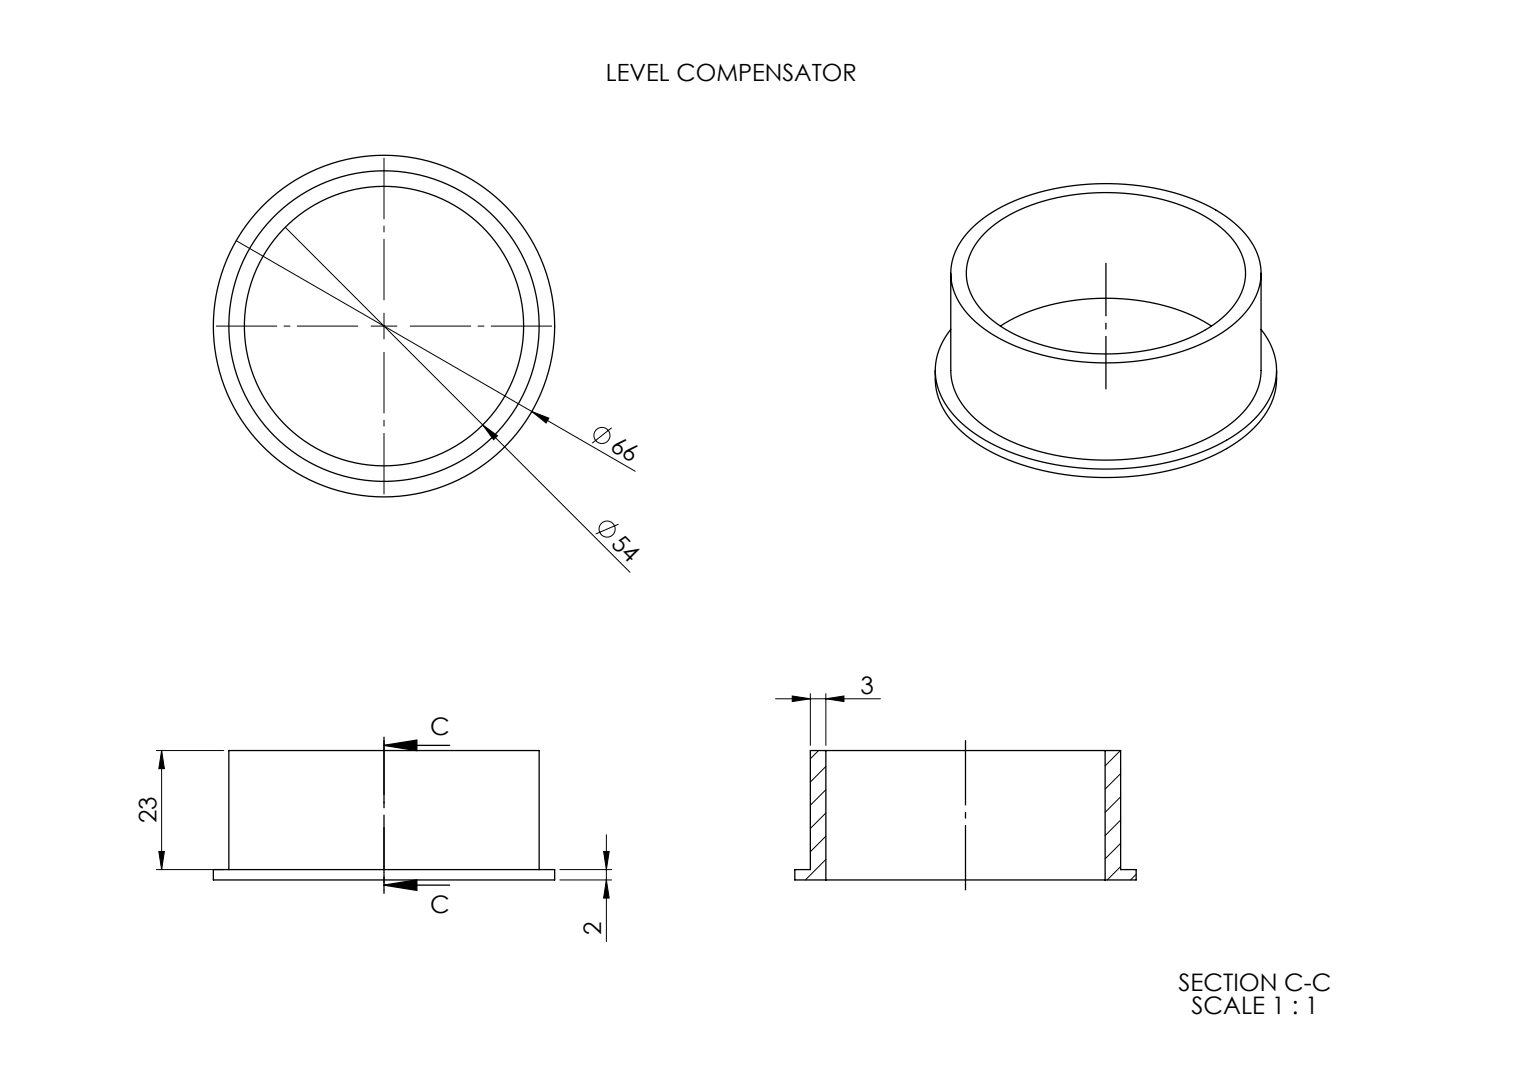
ISO-10303-21;
HEADER;
FILE_DESCRIPTION (('STEP AP214'),
    '1' );
FILE_NAME ('level compensator.step',
    '2026-10-02T18:08:48',
    ( '' ),
    ( '' ),
    'SwSTEP 2.0',
    'SolidWorks 2026',
    '' );
FILE_SCHEMA (( 'AUTOMOTIVE_DESIGN' ));
ENDSEC;

DATA;
#56=LINE ( 'NONE', #23253, #28638 ) ;
#123=ADVANCED_FACE ( 'NONE', ( #17350, #12018 ), #22832, .T. ) ;
#373=ORIENTED_EDGE ( 'NONE', *, *, #30700, .F. ) ;
#395=ORIENTED_EDGE ( 'NONE', *, *, #27322, .F. ) ;
#589=VECTOR ( 'NONE', #16460, 1000.000000000000000 ) ;
#693=CARTESIAN_POINT ( 'NONE',  ( 0.000000000000000000, -10.99999999999999645, 30.00000000000000000 ) ) ;
#907=CARTESIAN_POINT ( 'NONE',  ( 0.000000000000000000, -12.99999999999999822, 0.000000000000000000 ) ) ;
#1030=EDGE_CURVE ( 'NONE', #9545, #23066, #12266, .T. ) ;
#1166=AXIS2_PLACEMENT_3D ( 'NONE', #29236, #16220, #24104 ) ;
#1349=CARTESIAN_POINT ( 'NONE',  ( 4.041334437186266200E-15, -10.99999999999999645, 33.00000000000000000 ) ) ;
#1374=DIRECTION ( 'NONE',  ( 0.000000000000000000, -1.000000000000000000, 0.000000000000000000 ) ) ;
#1376=AXIS2_PLACEMENT_3D ( 'NONE', #6186, #27460, #21818 ) ;
#1489=CARTESIAN_POINT ( 'NONE',  ( 0.000000000000000000, 11.99999999999999645, 30.00000000000000000 ) ) ;
#1689=EDGE_CURVE ( 'NONE', #7405, #23066, #10874, .T. ) ;
#1782=EDGE_CURVE ( 'NONE', #20971, #6049, #18351, .T. ) ;
#1786=CARTESIAN_POINT ( 'NONE',  ( 4.041334437186266200E-15, -12.99999999999999822, 33.00000000000000000 ) ) ;
#1877=( LENGTH_UNIT ( ) NAMED_UNIT ( * ) SI_UNIT ( .MILLI., .METRE. ) );
#1908=ORIENTED_EDGE ( 'NONE', *, *, #1030, .T. ) ;
#1920=COLOUR_RGB ( '', 0.66274510, 0.83137255, 0.94901961) ;
#2047=FACE_BOUND ( 'NONE', #31107, .T. ) ;
#2135=DIRECTION ( 'NONE',  ( 0.000000000000000000, -1.000000000000000000, 0.000000000000000000 ) ) ;
#2140=DIRECTION ( 'NONE',  ( 0.000000000000000000, -1.000000000000000000, 0.000000000000000000 ) ) ;
#2313=DIRECTION ( 'NONE',  ( 0.000000000000000000, 0.000000000000000000, 1.000000000000000000 ) ) ;
#2455=ORIENTED_EDGE ( 'NONE', *, *, #27322, .T. ) ;
#2485=CYLINDRICAL_SURFACE ( 'NONE', #26189, 30.00000000000000000 ) ;
#2562=EDGE_LOOP ( 'NONE', ( #9167, #24597 ) ) ;
#2645=EDGE_LOOP ( 'NONE', ( #22385, #6844, #9366, #19276 ) ) ;
#2667=ADVANCED_FACE ( 'NONE', ( #20423, #2047 ), #4449, .F. ) ;
#2692=VERTEX_POINT ( 'NONE', #30872 ) ;
#2999=FACE_OUTER_BOUND ( 'NONE', #2645, .T. ) ;
#3170=CYLINDRICAL_SURFACE ( 'NONE', #1166, 27.00000000000000000 ) ;
#3270=ORIENTED_EDGE ( 'NONE', *, *, #13968, .F. ) ;
#3340=ADVANCED_FACE ( 'NONE', ( #23256 ), #2485, .T. ) ;
#3476=CARTESIAN_POINT ( 'NONE',  ( 0.000000000000000000, -10.99999999999999645, 0.000000000000000000 ) ) ;
#3549=DIRECTION ( 'NONE',  ( 0.000000000000000000, 0.000000000000000000, -1.000000000000000000 ) ) ;
#3597=MECHANICAL_DESIGN_GEOMETRIC_PRESENTATION_REPRESENTATION('',(#10711),#7987);
#3804=EDGE_CURVE ( 'NONE', #2692, #30646, #17443, .T. ) ;
#3810=DIRECTION ( 'NONE',  ( 0.000000000000000000, -1.000000000000000000, 0.000000000000000000 ) ) ;
#3928=AXIS2_PLACEMENT_3D ( 'NONE', #4887, #4714, #2313 ) ;
#4023=CARTESIAN_POINT ( 'NONE',  ( 0.000000000000000000, 11.99999999999999645, 0.000000000000000000 ) ) ;
#4037=CIRCLE ( 'NONE', #16120, 33.00000000000000000 ) ;
#4449=PLANE ( 'NONE',  #17391 ) ;
#4469=EDGE_LOOP ( 'NONE', ( #23792, #1908 ) ) ;
#4548=DIRECTION ( 'NONE',  ( 0.000000000000000000, 0.000000000000000000, -1.000000000000000000 ) ) ;
#4605=FACE_BOUND ( 'NONE', #20807, .T. ) ;
#4714=DIRECTION ( 'NONE',  ( -0.000000000000000000, 1.000000000000000000, -0.000000000000000000 ) ) ;
#4884=CARTESIAN_POINT ( 'NONE',  ( 0.000000000000000000, -12.99999999999999822, 0.000000000000000000 ) ) ;
#4887=CARTESIAN_POINT ( 'NONE',  ( 0.000000000000000000, -12.99999999999999822, 0.000000000000000000 ) ) ;
#4955=EDGE_CURVE ( 'NONE', #6049, #20971, #26216, .T. ) ;
#5149=CLOSED_SHELL ( 'NONE', ( #16079, #9447, #29369, #3340, #123, #2667, #9646, #28558, #31037 ) ) ;
#5223=ORIENTED_EDGE ( 'NONE', *, *, #1782, .F. ) ;
#5228=FACE_OUTER_BOUND ( 'NONE', #11535, .T. ) ;
#5566=DIRECTION ( 'NONE',  ( -0.000000000000000000, 1.000000000000000000, -0.000000000000000000 ) ) ;
#5696=AXIS2_PLACEMENT_3D ( 'NONE', #28118, #27437, #33431 ) ;
#6011=ORIENTED_EDGE ( 'NONE', *, *, #25422, .F. ) ;
#6033=DIRECTION ( 'NONE',  ( 0.000000000000000000, -1.000000000000000000, 0.000000000000000000 ) ) ;
#6049=VERTEX_POINT ( 'NONE', #17755 ) ;
#6163=PRODUCT_DEFINITION ( 'UNKNOWN', '', #13174, #6504 ) ;
#6186=CARTESIAN_POINT ( 'NONE',  ( 0.000000000000000000, 0.000000000000000000, 0.000000000000000000 ) ) ;
#6249=CIRCLE ( 'NONE', #27606, 30.00000000000000000 ) ;
#6504=PRODUCT_DEFINITION_CONTEXT ( 'detailed design', #21934, 'design' ) ;
#6669=DIRECTION ( 'NONE',  ( 1.000000000000000000, 0.000000000000000000, 0.000000000000000000 ) ) ;
#6844=ORIENTED_EDGE ( 'NONE', *, *, #28947, .T. ) ;
#6912=ORIENTED_EDGE ( 'NONE', *, *, #14411, .T. ) ;
#7039=VERTEX_POINT ( 'NONE', #1349 ) ;
#7285=FACE_OUTER_BOUND ( 'NONE', #32956, .T. ) ;
#7321=CIRCLE ( 'NONE', #29774, 27.00000000000000000 ) ;
#7376=SURFACE_SIDE_STYLE ('',( #10130 ) ) ;
#7405=VERTEX_POINT ( 'NONE', #23151 ) ;
#7541=DIRECTION ( 'NONE',  ( 0.000000000000000000, -0.000000000000000000, -1.000000000000000000 ) ) ;
#7828=EDGE_LOOP ( 'NONE', ( #373, #24739 ) ) ;
#7973=CARTESIAN_POINT ( 'NONE',  ( 0.000000000000000000, -12.99999999999999822, 0.000000000000000000 ) ) ;
#7987=( GEOMETRIC_REPRESENTATION_CONTEXT ( 3 ) GLOBAL_UNCERTAINTY_ASSIGNED_CONTEXT ( ( #18089 ) ) GLOBAL_UNIT_ASSIGNED_CONTEXT ( ( #1877, #9779, #20430 ) ) REPRESENTATION_CONTEXT ( 'NONE', 'WORKASPACE' ) );
#8140=( NAMED_UNIT ( * ) SI_UNIT ( $, .STERADIAN. ) SOLID_ANGLE_UNIT ( ) );
#8214=EDGE_CURVE ( 'NONE', #30646, #2692, #32934, .T. ) ;
#8281=DIRECTION ( 'NONE',  ( 0.000000000000000000, -1.000000000000000000, 0.000000000000000000 ) ) ;
#8289=ORIENTED_EDGE ( 'NONE', *, *, #30841, .T. ) ;
#8312=COLOUR_RGB ( '', 0.66274510, 0.83137255, 0.94901961) ;
#8662=ORIENTED_EDGE ( 'NONE', *, *, #1689, .F. ) ;
#8792=VERTEX_POINT ( 'NONE', #1489 ) ;
#8835=ORIENTED_EDGE ( 'NONE', *, *, #16099, .F. ) ;
#9133=AXIS2_PLACEMENT_3D ( 'NONE', #22331, #18929, #16352 ) ;
#9167=ORIENTED_EDGE ( 'NONE', *, *, #30966, .F. ) ;
#9234=CARTESIAN_POINT ( 'NONE',  ( 0.000000000000000000, -10.99999999999999645, 0.000000000000000000 ) ) ;
#9366=ORIENTED_EDGE ( 'NONE', *, *, #21542, .T. ) ;
#9369=ORIENTED_EDGE ( 'NONE', *, *, #1782, .T. ) ;
#9447=ADVANCED_FACE ( 'NONE', ( #7285 ), #17769, .F. ) ;
#9471=VECTOR ( 'NONE', #33843, 1000.000000000000000 ) ;
#9545=VERTEX_POINT ( 'NONE', #1786 ) ;
#9552=MANIFOLD_SOLID_BREP ( 'Extrude-Thin2', #5149 ) ;
#9646=ADVANCED_FACE ( 'NONE', ( #2999 ), #3170, .F. ) ;
#9683=CIRCLE ( 'NONE', #9133, 30.00000000000000000 ) ;
#9779=( NAMED_UNIT ( * ) PLANE_ANGLE_UNIT ( ) SI_UNIT ( $, .RADIAN. ) );
#9792=CARTESIAN_POINT ( 'NONE',  ( 0.000000000000000000, -12.99999999999999822, 0.000000000000000000 ) ) ;
#9928=DIRECTION ( 'NONE',  ( 0.000000000000000000, -1.000000000000000000, 0.000000000000000000 ) ) ;
#10130=SURFACE_STYLE_FILL_AREA ( #20612 ) ;
#10193=UNCERTAINTY_MEASURE_WITH_UNIT (LENGTH_MEASURE( 1.000000000000000082E-05 ), #10720, 'distance_accuracy_value', 'NONE');
#10380=CYLINDRICAL_SURFACE ( 'NONE', #33589, 33.00000000000000000 ) ;
#10448=PRODUCT_DEFINITION_SHAPE ( 'NONE', 'NONE',  #6163 ) ;
#10711=STYLED_ITEM ( 'NONE', ( #17860 ), #22997 ) ;
#10720=( LENGTH_UNIT ( ) NAMED_UNIT ( * ) SI_UNIT ( .MILLI., .METRE. ) );
#10750=ORIENTED_EDGE ( 'NONE', *, *, #8214, .T. ) ;
#10874=LINE ( 'NONE', #33873, #22682 ) ;
#11303=CARTESIAN_POINT ( 'NONE',  ( 0.000000000000000000, -12.99999999999999822, 27.00000000000000000 ) ) ;
#11535=EDGE_LOOP ( 'NONE', ( #395, #8289, #29593, #27174 ) ) ;
#11648=CARTESIAN_POINT ( 'NONE',  ( 0.000000000000000000, -12.99999999999999822, 0.000000000000000000 ) ) ;
#11724=AXIS2_PLACEMENT_3D ( 'NONE', #9792, #1374, #20268 ) ;
#11852=FACE_OUTER_BOUND ( 'NONE', #15049, .T. ) ;
#12018=FACE_OUTER_BOUND ( 'NONE', #4469, .T. ) ;
#12194=VECTOR ( 'NONE', #22625, 1000.000000000000000 ) ;
#12248=EDGE_LOOP ( 'NONE', ( #3270, #5223, #16778, #16744 ) ) ;
#12266=CIRCLE ( 'NONE', #19941, 33.00000000000000000 ) ;
#12735=ORIENTED_EDGE ( 'NONE', *, *, #21542, .F. ) ;
#12846=DIRECTION ( 'NONE',  ( -0.000000000000000000, 1.000000000000000000, -0.000000000000000000 ) ) ;
#13122=PRESENTATION_STYLE_ASSIGNMENT (( #18629 ) ) ;
#13174=PRODUCT_DEFINITION_FORMATION_WITH_SPECIFIED_SOURCE ( 'ANY', '', #20871, .NOT_KNOWN. ) ;
#13500=ORIENTED_EDGE ( 'NONE', *, *, #28224, .F. ) ;
#13802=( NAMED_UNIT ( * ) PLANE_ANGLE_UNIT ( ) SI_UNIT ( $, .RADIAN. ) );
#13875=VECTOR ( 'NONE', #12846, 1000.000000000000000 ) ;
#13947=DIRECTION ( 'NONE',  ( 0.000000000000000000, 0.000000000000000000, -1.000000000000000000 ) ) ;
#13968=EDGE_CURVE ( 'NONE', #6049, #16699, #20061, .T. ) ;
#14235=CARTESIAN_POINT ( 'NONE',  ( 0.000000000000000000, 11.99999999999999645, 27.00000000000000000 ) ) ;
#14304=DIRECTION ( 'NONE',  ( 0.000000000000000000, -1.000000000000000000, 0.000000000000000000 ) ) ;
#14411=EDGE_CURVE ( 'NONE', #29507, #2692, #26058, .T. ) ;
#14847=FILL_AREA_STYLE ('',( #33890 ) ) ;
#14909=DIRECTION ( 'NONE',  ( 1.000000000000000000, 0.000000000000000000, 0.000000000000000000 ) ) ;
#14934=SURFACE_STYLE_USAGE ( .BOTH. , #7376 ) ;
#15025=AXIS2_PLACEMENT_3D ( 'NONE', #907, #14304, #19126 ) ;
#15049=EDGE_LOOP ( 'NONE', ( #30960, #2455, #6011, #8662 ) ) ;
#15145=ORIENTED_EDGE ( 'NONE', *, *, #16099, .T. ) ;
#15150=DIRECTION ( 'NONE',  ( 0.000000000000000000, -1.000000000000000000, 0.000000000000000000 ) ) ;
#15188=DIRECTION ( 'NONE',  ( 0.000000000000000000, -1.000000000000000000, 0.000000000000000000 ) ) ;
#15279=SHAPE_REPRESENTATION_RELATIONSHIP ( 'NONE' , 'NONE' ,  #15301, #22997 ) ;
#15301=SHAPE_REPRESENTATION ( 'level compensator', ( #1376 ), #21134 ) ;
#15367=CARTESIAN_POINT ( 'NONE',  ( 0.000000000000000000, -10.99999999999999645, 0.000000000000000000 ) ) ;
#16079=ADVANCED_FACE ( 'NONE', ( #11852 ), #32611, .T. ) ;
#16099=EDGE_CURVE ( 'NONE', #16699, #8792, #9683, .T. ) ;
#16120=AXIS2_PLACEMENT_3D ( 'NONE', #9234, #9928, #6669 ) ;
#16220=DIRECTION ( 'NONE',  ( -0.000000000000000000, 1.000000000000000000, -0.000000000000000000 ) ) ;
#16352=DIRECTION ( 'NONE',  ( 0.000000000000000000, 0.000000000000000000, -1.000000000000000000 ) ) ;
#16460=DIRECTION ( 'NONE',  ( -0.000000000000000000, 1.000000000000000000, -0.000000000000000000 ) ) ;
#16689=AXIS2_PLACEMENT_3D ( 'NONE', #3476, #3810, #13947 ) ;
#16699=VERTEX_POINT ( 'NONE', #29831 ) ;
#16744=ORIENTED_EDGE ( 'NONE', *, *, #25075, .T. ) ;
#16778=ORIENTED_EDGE ( 'NONE', *, *, #28224, .T. ) ;
#17068=ORIENTED_EDGE ( 'NONE', *, *, #25075, .F. ) ;
#17088=STYLED_ITEM ( 'NONE', ( #13122 ), #9552 ) ;
#17350=FACE_BOUND ( 'NONE', #7828, .T. ) ;
#17391=AXIS2_PLACEMENT_3D ( 'NONE', #23339, #33801, #7541 ) ;
#17443=CIRCLE ( 'NONE', #33882, 27.00000000000000000 ) ;
#17657=PLANE ( 'NONE',  #5696 ) ;
#17755=CARTESIAN_POINT ( 'NONE',  ( 3.673940397442059178E-15, -10.99999999999999645, -30.00000000000000000 ) ) ;
#17761=EDGE_LOOP ( 'NONE', ( #33796, #24378, #15145, #13500 ) ) ;
#17769=CYLINDRICAL_SURFACE ( 'NONE', #3928, 27.00000000000000000 ) ;
#17860=PRESENTATION_STYLE_ASSIGNMENT (( #14934 ) ) ;
#18089=UNCERTAINTY_MEASURE_WITH_UNIT (LENGTH_MEASURE( 1.000000000000000082E-05 ), #1877, 'distance_accuracy_value', 'NONE');
#18111=DIRECTION ( 'NONE',  ( 0.000000000000000000, 0.000000000000000000, -1.000000000000000000 ) ) ;
#18172=DIRECTION ( 'NONE',  ( 0.000000000000000000, -1.000000000000000000, 0.000000000000000000 ) ) ;
#18210=MECHANICAL_DESIGN_GEOMETRIC_PRESENTATION_REPRESENTATION('',(#17088),#22563);
#18351=CIRCLE ( 'NONE', #16689, 30.00000000000000000 ) ;
#18479=AXIS2_PLACEMENT_3D ( 'NONE', #29530, #6033, #19589 ) ;
#18629=SURFACE_STYLE_USAGE ( .BOTH. , #26836 ) ;
#18888=DIRECTION ( 'NONE',  ( 0.000000000000000000, -1.000000000000000000, 0.000000000000000000 ) ) ;
#18929=DIRECTION ( 'NONE',  ( 0.000000000000000000, -1.000000000000000000, 0.000000000000000000 ) ) ;
#18960=SURFACE_STYLE_FILL_AREA ( #14847 ) ;
#19126=DIRECTION ( 'NONE',  ( 1.000000000000000000, 0.000000000000000000, 0.000000000000000000 ) ) ;
#19270=AXIS2_PLACEMENT_3D ( 'NONE', #4023, #28390, #33881 ) ;
#19276=ORIENTED_EDGE ( 'NONE', *, *, #3804, .F. ) ;
#19342=DIRECTION ( 'NONE',  ( 0.000000000000000000, -1.000000000000000000, 0.000000000000000000 ) ) ;
#19365=AXIS2_PLACEMENT_3D ( 'NONE', #33637, #22656, #22829 ) ;
#19589=DIRECTION ( 'NONE',  ( 0.000000000000000000, 0.000000000000000000, -1.000000000000000000 ) ) ;
#19770=EDGE_LOOP ( 'NONE', ( #17068, #8835 ) ) ;
#19941=AXIS2_PLACEMENT_3D ( 'NONE', #23315, #18172, #20752 ) ;
#20061=LINE ( 'NONE', #27269, #12194 ) ;
#20062=CARTESIAN_POINT ( 'NONE',  ( 0.000000000000000000, -10.99999999999999645, 0.000000000000000000 ) ) ;
#20187=APPLICATION_CONTEXT ( 'automotive_design' ) ;
#20268=DIRECTION ( 'NONE',  ( 0.000000000000000000, -0.000000000000000000, -1.000000000000000000 ) ) ;
#20423=FACE_OUTER_BOUND ( 'NONE', #19770, .T. ) ;
#20430=( NAMED_UNIT ( * ) SI_UNIT ( $, .STERADIAN. ) SOLID_ANGLE_UNIT ( ) );
#20492=UNCERTAINTY_MEASURE_WITH_UNIT (LENGTH_MEASURE( 1.000000000000000082E-05 ), #30879, 'distance_accuracy_value', 'NONE');
#20500=CIRCLE ( 'NONE', #22659, 33.00000000000000000 ) ;
#20612=FILL_AREA_STYLE ('',( #30360 ) ) ;
#20752=DIRECTION ( 'NONE',  ( 1.000000000000000000, 0.000000000000000000, 0.000000000000000000 ) ) ;
#20807=EDGE_LOOP ( 'NONE', ( #9369, #23413 ) ) ;
#20857=DIRECTION ( 'NONE',  ( 0.000000000000000000, 0.000000000000000000, 1.000000000000000000 ) ) ;
#20871=PRODUCT ( 'level compensator', 'level compensator', '', ( #26382 ) ) ;
#20971=VERTEX_POINT ( 'NONE', #693 ) ;
#20995=CARTESIAN_POINT ( 'NONE',  ( 0.000000000000000000, -12.99999999999999822, 27.00000000000000000 ) ) ;
#21134=( GEOMETRIC_REPRESENTATION_CONTEXT ( 3 ) GLOBAL_UNCERTAINTY_ASSIGNED_CONTEXT ( ( #20492 ) ) GLOBAL_UNIT_ASSIGNED_CONTEXT ( ( #30879, #33283, #23169 ) ) REPRESENTATION_CONTEXT ( 'NONE', 'WORKASPACE' ) );
#21542=EDGE_CURVE ( 'NONE', #25961, #30646, #32056, .T. ) ;
#21818=DIRECTION ( 'NONE',  ( 1.000000000000000000, 0.000000000000000000, 0.000000000000000000 ) ) ;
#21934=APPLICATION_CONTEXT ( 'automotive_design' ) ;
#22131=DIRECTION ( 'NONE',  ( 1.000000000000000000, 0.000000000000000000, 0.000000000000000000 ) ) ;
#22331=CARTESIAN_POINT ( 'NONE',  ( 0.000000000000000000, 11.99999999999999645, 0.000000000000000000 ) ) ;
#22385=ORIENTED_EDGE ( 'NONE', *, *, #14411, .F. ) ;
#22563=( GEOMETRIC_REPRESENTATION_CONTEXT ( 3 ) GLOBAL_UNCERTAINTY_ASSIGNED_CONTEXT ( ( #10193 ) ) GLOBAL_UNIT_ASSIGNED_CONTEXT ( ( #10720, #13802, #8140 ) ) REPRESENTATION_CONTEXT ( 'NONE', 'WORKASPACE' ) );
#22566=DIRECTION ( 'NONE',  ( 0.000000000000000000, -1.000000000000000000, 0.000000000000000000 ) ) ;
#22625=DIRECTION ( 'NONE',  ( -0.000000000000000000, 1.000000000000000000, -0.000000000000000000 ) ) ;
#22636=AXIS2_PLACEMENT_3D ( 'NONE', #7973, #2140, #31144 ) ;
#22656=DIRECTION ( 'NONE',  ( -0.000000000000000000, 1.000000000000000000, -0.000000000000000000 ) ) ;
#22659=AXIS2_PLACEMENT_3D ( 'NONE', #20062, #22972, #14909 ) ;
#22682=VECTOR ( 'NONE', #8281, 1000.000000000000000 ) ;
#22743=CARTESIAN_POINT ( 'NONE',  ( 0.000000000000000000, 11.99999999999999645, 0.000000000000000000 ) ) ;
#22829=DIRECTION ( 'NONE',  ( 0.000000000000000000, 0.000000000000000000, 1.000000000000000000 ) ) ;
#22832=PLANE ( 'NONE',  #11724 ) ;
#22854=ORIENTED_EDGE ( 'NONE', *, *, #3804, .T. ) ;
#22972=DIRECTION ( 'NONE',  ( 0.000000000000000000, -1.000000000000000000, 0.000000000000000000 ) ) ;
#22997=ADVANCED_BREP_SHAPE_REPRESENTATION ( '', ( #9552, #1376 ), #21134 ) ;
#23066=VERTEX_POINT ( 'NONE', #26554 ) ;
#23138=CARTESIAN_POINT ( 'NONE',  ( 3.306546357697853733E-15, -12.99999999999999822, -27.00000000000000000 ) ) ;
#23151=CARTESIAN_POINT ( 'NONE',  ( 0.000000000000000000, -10.99999999999999645, -33.00000000000000000 ) ) ;
#23169=( NAMED_UNIT ( * ) SI_UNIT ( $, .STERADIAN. ) SOLID_ANGLE_UNIT ( ) );
#23241=CIRCLE ( 'NONE', #15025, 33.00000000000000000 ) ;
#23253=CARTESIAN_POINT ( 'NONE',  ( 4.041334437186266200E-15, -10.99999999999999645, 33.00000000000000000 ) ) ;
#23256=FACE_OUTER_BOUND ( 'NONE', #12248, .T. ) ;
#23315=CARTESIAN_POINT ( 'NONE',  ( 0.000000000000000000, -12.99999999999999822, 0.000000000000000000 ) ) ;
#23339=CARTESIAN_POINT ( 'NONE',  ( 0.000000000000000000, 11.99999999999999645, 0.000000000000000000 ) ) ;
#23380=LINE ( 'NONE', #28852, #9471 ) ;
#23413=ORIENTED_EDGE ( 'NONE', *, *, #4955, .T. ) ;
#23792=ORIENTED_EDGE ( 'NONE', *, *, #25422, .T. ) ;
#24104=DIRECTION ( 'NONE',  ( 0.000000000000000000, 0.000000000000000000, 1.000000000000000000 ) ) ;
#24134=ORIENTED_EDGE ( 'NONE', *, *, #30700, .T. ) ;
#24378=ORIENTED_EDGE ( 'NONE', *, *, #13968, .T. ) ;
#24597=ORIENTED_EDGE ( 'NONE', *, *, #30841, .F. ) ;
#24739=ORIENTED_EDGE ( 'NONE', *, *, #28947, .F. ) ;
#25075=EDGE_CURVE ( 'NONE', #8792, #16699, #6249, .T. ) ;
#25405=CYLINDRICAL_SURFACE ( 'NONE', #19365, 30.00000000000000000 ) ;
#25422=EDGE_CURVE ( 'NONE', #23066, #9545, #23241, .T. ) ;
#25614=DIRECTION ( 'NONE',  ( 1.000000000000000000, 0.000000000000000000, 0.000000000000000000 ) ) ;
#25745=FACE_OUTER_BOUND ( 'NONE', #17761, .T. ) ;
#25961=VERTEX_POINT ( 'NONE', #20995 ) ;
#26058=LINE ( 'NONE', #23138, #13875 ) ;
#26189=AXIS2_PLACEMENT_3D ( 'NONE', #4884, #5566, #20857 ) ;
#26216=CIRCLE ( 'NONE', #31133, 30.00000000000000000 ) ;
#26319=ORIENTED_EDGE ( 'NONE', *, *, #8214, .F. ) ;
#26382=PRODUCT_CONTEXT ( 'NONE', #20187, 'mechanical' ) ;
#26554=CARTESIAN_POINT ( 'NONE',  ( 0.000000000000000000, -12.99999999999999822, -33.00000000000000000 ) ) ;
#26731=CARTESIAN_POINT ( 'NONE',  ( 0.000000000000000000, -10.99999999999999645, 0.000000000000000000 ) ) ;
#26836=SURFACE_SIDE_STYLE ('',( #18960 ) ) ;
#27174=ORIENTED_EDGE ( 'NONE', *, *, #1030, .F. ) ;
#27269=CARTESIAN_POINT ( 'NONE',  ( 3.673940397442059178E-15, -12.99999999999999822, -30.00000000000000000 ) ) ;
#27322=EDGE_CURVE ( 'NONE', #7039, #9545, #56, .T. ) ;
#27437=DIRECTION ( 'NONE',  ( 0.000000000000000000, -1.000000000000000000, 0.000000000000000000 ) ) ;
#27460=DIRECTION ( 'NONE',  ( 0.000000000000000000, 0.000000000000000000, 1.000000000000000000 ) ) ;
#27500=CARTESIAN_POINT ( 'NONE',  ( 0.000000000000000000, 11.99999999999999645, 0.000000000000000000 ) ) ;
#27559=CIRCLE ( 'NONE', #22636, 27.00000000000000000 ) ;
#27606=AXIS2_PLACEMENT_3D ( 'NONE', #22743, #22566, #4548 ) ;
#28118=CARTESIAN_POINT ( 'NONE',  ( 0.000000000000000000, -10.99999999999999645, 0.000000000000000000 ) ) ;
#28224=EDGE_CURVE ( 'NONE', #20971, #8792, #23380, .T. ) ;
#28318=CARTESIAN_POINT ( 'NONE',  ( 3.306546357697853733E-15, -12.99999999999999822, -27.00000000000000000 ) ) ;
#28390=DIRECTION ( 'NONE',  ( 0.000000000000000000, -1.000000000000000000, 0.000000000000000000 ) ) ;
#28558=ADVANCED_FACE ( 'NONE', ( #5228 ), #10380, .T. ) ;
#28604=SHAPE_DEFINITION_REPRESENTATION ( #10448, #15301 ) ;
#28638=VECTOR ( 'NONE', #15188, 1000.000000000000000 ) ;
#28852=CARTESIAN_POINT ( 'NONE',  ( 0.000000000000000000, -12.99999999999999822, 30.00000000000000000 ) ) ;
#28947=EDGE_CURVE ( 'NONE', #29507, #25961, #27559, .T. ) ;
#29236=CARTESIAN_POINT ( 'NONE',  ( 0.000000000000000000, -12.99999999999999822, 0.000000000000000000 ) ) ;
#29369=ADVANCED_FACE ( 'NONE', ( #25745 ), #25405, .T. ) ;
#29507=VERTEX_POINT ( 'NONE', #28318 ) ;
#29530=CARTESIAN_POINT ( 'NONE',  ( 0.000000000000000000, -10.99999999999999645, 0.000000000000000000 ) ) ;
#29593=ORIENTED_EDGE ( 'NONE', *, *, #1689, .T. ) ;
#29774=AXIS2_PLACEMENT_3D ( 'NONE', #11648, #18888, #22131 ) ;
#29831=CARTESIAN_POINT ( 'NONE',  ( 3.673940397442059178E-15, 11.99999999999999645, -30.00000000000000000 ) ) ;
#30360=FILL_AREA_STYLE_COLOUR ( '', #1920 ) ;
#30646=VERTEX_POINT ( 'NONE', #14235 ) ;
#30700=EDGE_CURVE ( 'NONE', #25961, #29507, #7321, .T. ) ;
#30841=EDGE_CURVE ( 'NONE', #7039, #7405, #4037, .T. ) ;
#30872=CARTESIAN_POINT ( 'NONE',  ( 3.306546357697853733E-15, 11.99999999999999645, -27.00000000000000000 ) ) ;
#30879=( LENGTH_UNIT ( ) NAMED_UNIT ( * ) SI_UNIT ( .MILLI., .METRE. ) );
#30960=ORIENTED_EDGE ( 'NONE', *, *, #30966, .T. ) ;
#30966=EDGE_CURVE ( 'NONE', #7405, #7039, #20500, .T. ) ;
#31037=ADVANCED_FACE ( 'NONE', ( #4605, #33256 ), #17657, .F. ) ;
#31107=EDGE_LOOP ( 'NONE', ( #10750, #22854 ) ) ;
#31133=AXIS2_PLACEMENT_3D ( 'NONE', #26731, #19342, #3549 ) ;
#31144=DIRECTION ( 'NONE',  ( 1.000000000000000000, 0.000000000000000000, 0.000000000000000000 ) ) ;
#32056=LINE ( 'NONE', #11303, #589 ) ;
#32611=CYLINDRICAL_SURFACE ( 'NONE', #18479, 33.00000000000000000 ) ;
#32934=CIRCLE ( 'NONE', #19270, 27.00000000000000000 ) ;
#32956=EDGE_LOOP ( 'NONE', ( #24134, #6912, #26319, #12735 ) ) ;
#33256=FACE_OUTER_BOUND ( 'NONE', #2562, .T. ) ;
#33283=( NAMED_UNIT ( * ) PLANE_ANGLE_UNIT ( ) SI_UNIT ( $, .RADIAN. ) );
#33431=DIRECTION ( 'NONE',  ( 0.000000000000000000, -0.000000000000000000, -1.000000000000000000 ) ) ;
#33589=AXIS2_PLACEMENT_3D ( 'NONE', #15367, #2135, #18111 ) ;
#33637=CARTESIAN_POINT ( 'NONE',  ( 0.000000000000000000, -12.99999999999999822, 0.000000000000000000 ) ) ;
#33796=ORIENTED_EDGE ( 'NONE', *, *, #4955, .F. ) ;
#33801=DIRECTION ( 'NONE',  ( 0.000000000000000000, -1.000000000000000000, 0.000000000000000000 ) ) ;
#33843=DIRECTION ( 'NONE',  ( -0.000000000000000000, 1.000000000000000000, -0.000000000000000000 ) ) ;
#33873=CARTESIAN_POINT ( 'NONE',  ( 0.000000000000000000, -10.99999999999999645, -33.00000000000000000 ) ) ;
#33881=DIRECTION ( 'NONE',  ( 1.000000000000000000, 0.000000000000000000, 0.000000000000000000 ) ) ;
#33882=AXIS2_PLACEMENT_3D ( 'NONE', #27500, #15150, #25614 ) ;
#33890=FILL_AREA_STYLE_COLOUR ( '', #8312 ) ;
ENDSEC;
END-ISO-10303-21;
